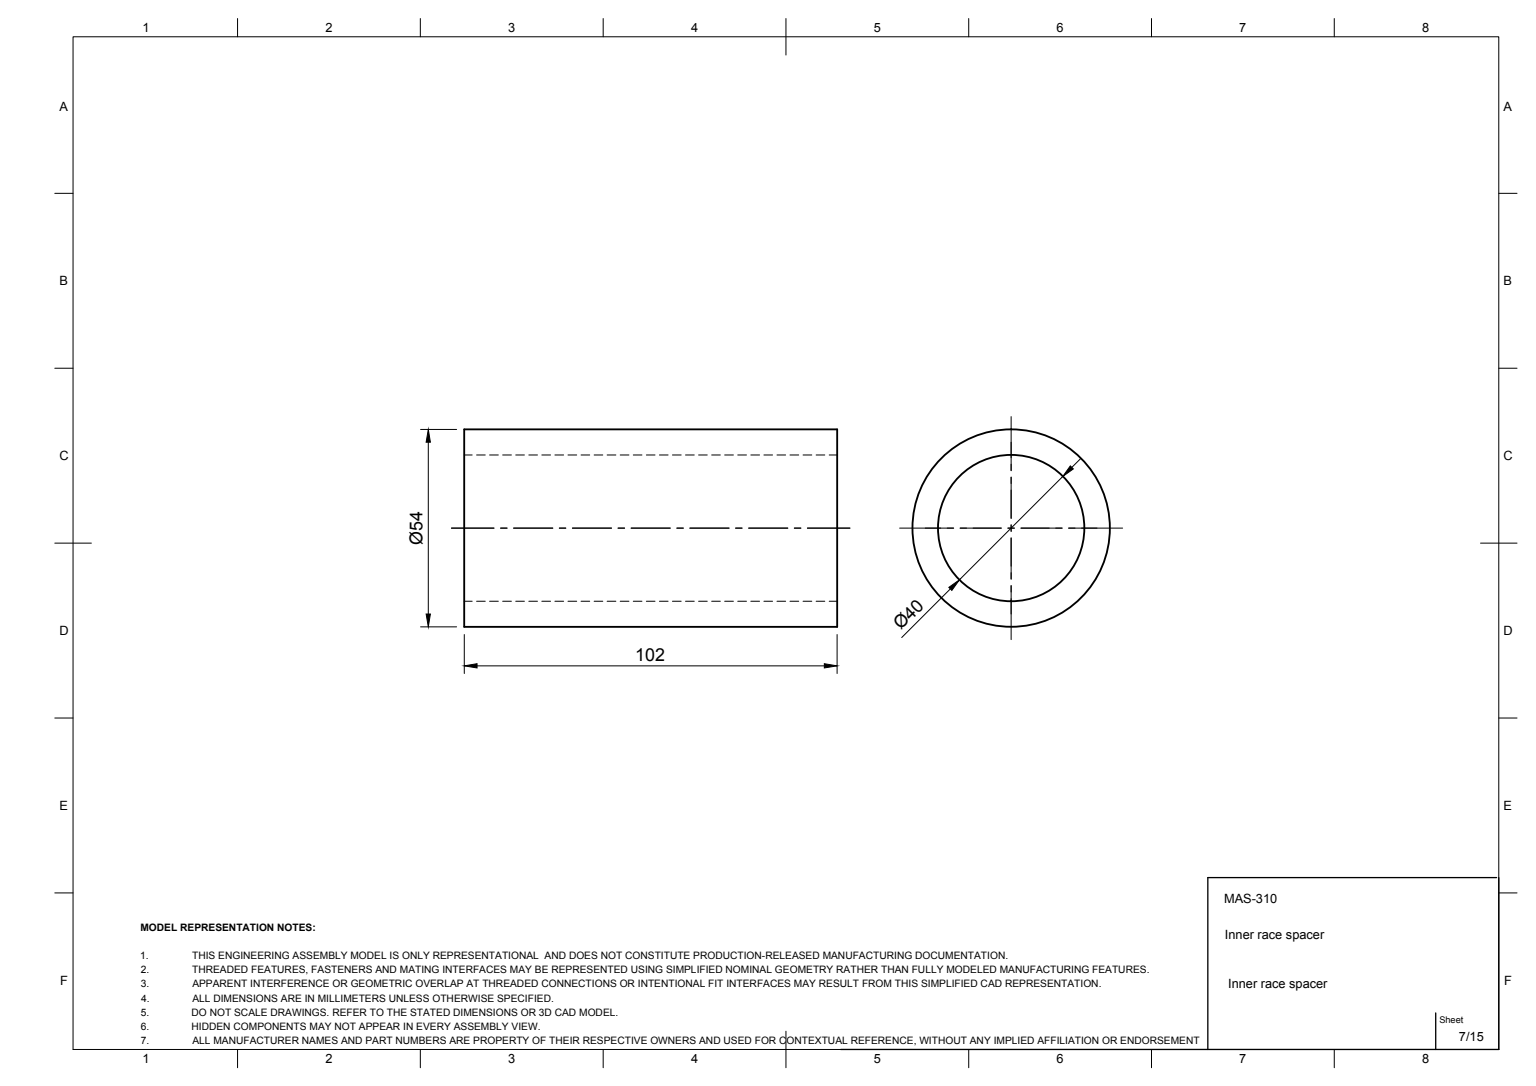
ISO-10303-21;
HEADER;
/* Generated by software containing ST-Developer
 * from STEP Tools, Inc. (www.steptools.com) 
 */

FILE_DESCRIPTION(
/* description */ ('Independent30mm screw-fed quill/spindle unit with16mm straight tool s
ocket, radial set screw, native reusable open ball bearings, retained 
inner/outer race stacks, keyed quill guide and M12x1.75 fine feed. Ext
ernal moving drive and tool not included. Ideal cage orbital links; in
dividual ball spin, force and preload not simulated. No drilling capac
ity, runout, speed, torque, load, life or machine safety rating.'),
/* implementation_level */ '2;1');

FILE_NAME(
/* name */ 'Inner race spacer.step',
/* time_stamp */ '2026-11-08T18:59:42-08:00',
/* author */ (''),
/* organization */ (''),
/* preprocessor_version */ 'ST-DEVELOPER v20.2',
/* originating_system */ 'Autodesk Translation Framework v15.17.0.0',
/* authorisation */ '');

FILE_SCHEMA (('AUTOMOTIVE_DESIGN { 1 0 10303 214 3 1 1 }'));
ENDSEC;

DATA;
#10=MECHANICAL_DESIGN_GEOMETRIC_PRESENTATION_REPRESENTATION('',(#1595),#63898);
#1559=SHAPE_REPRESENTATION_RELATIONSHIP('SRR','None',#63998,#1577);
#1577=ADVANCED_BREP_SHAPE_REPRESENTATION('',(#1613),#63883);
#1595=STYLED_ITEM('',(#64097),#1613);
#1613=MANIFOLD_SOLID_BREP('Body1',#15481);
#1669=FACE_BOUND('',#4012,.T.);
#1670=FACE_BOUND('',#4014,.T.);
#2106=CYLINDRICAL_SURFACE('',#16269,20.);
#2107=CYLINDRICAL_SURFACE('',#16272,27.);
#2499=CIRCLE('',#16270,20.);
#2500=CIRCLE('',#16271,20.);
#2501=CIRCLE('',#16273,27.);
#2502=CIRCLE('',#16274,27.);
#3130=FACE_OUTER_BOUND('',#4009,.T.);
#3131=FACE_OUTER_BOUND('',#4010,.T.);
#3132=FACE_OUTER_BOUND('',#4011,.T.);
#3133=FACE_OUTER_BOUND('',#4013,.T.);
#4009=EDGE_LOOP('',(#12496,#12497,#12498,#12499));
#4010=EDGE_LOOP('',(#12500,#12501,#12502,#12503));
#4011=EDGE_LOOP('',(#12504));
#4012=EDGE_LOOP('',(#12505));
#4013=EDGE_LOOP('',(#12506));
#4014=EDGE_LOOP('',(#12507));
#4856=LINE('',#46760,#5619);
#4857=LINE('',#46766,#5620);
#5619=VECTOR('',#18444,20.);
#5620=VECTOR('',#18451,27.);
#6832=VERTEX_POINT('',#46757);
#6833=VERTEX_POINT('',#46759);
#6834=VERTEX_POINT('',#46763);
#6835=VERTEX_POINT('',#46765);
#8837=EDGE_CURVE('',#6832,#6832,#2499,.T.);
#8838=EDGE_CURVE('',#6832,#6833,#4856,.T.);
#8839=EDGE_CURVE('',#6833,#6833,#2500,.T.);
#8840=EDGE_CURVE('',#6834,#6834,#2501,.T.);
#8841=EDGE_CURVE('',#6834,#6835,#4857,.T.);
#8842=EDGE_CURVE('',#6835,#6835,#2502,.T.);
#12496=ORIENTED_EDGE('',*,*,#8837,.F.);
#12497=ORIENTED_EDGE('',*,*,#8838,.T.);
#12498=ORIENTED_EDGE('',*,*,#8839,.T.);
#12499=ORIENTED_EDGE('',*,*,#8838,.F.);
#12500=ORIENTED_EDGE('',*,*,#8840,.F.);
#12501=ORIENTED_EDGE('',*,*,#8841,.T.);
#12502=ORIENTED_EDGE('',*,*,#8842,.T.);
#12503=ORIENTED_EDGE('',*,*,#8841,.F.);
#12504=ORIENTED_EDGE('',*,*,#8840,.T.);
#12505=ORIENTED_EDGE('',*,*,#8837,.T.);
#12506=ORIENTED_EDGE('',*,*,#8842,.F.);
#12507=ORIENTED_EDGE('',*,*,#8839,.F.);
#14569=PLANE('',#16275);
#14570=PLANE('',#16276);
#15110=ADVANCED_FACE('',(#3130),#2106,.F.);
#15111=ADVANCED_FACE('',(#3131),#2107,.T.);
#15112=ADVANCED_FACE('',(#3132,#1669),#14569,.T.);
#15113=ADVANCED_FACE('',(#3133,#1670),#14570,.F.);
#15481=CLOSED_SHELL('',(#15110,#15111,#15112,#15113));
#16268=AXIS2_PLACEMENT_3D('',#46755,#18438,#18439);
#16269=AXIS2_PLACEMENT_3D('',#46756,#18440,#18441);
#16270=AXIS2_PLACEMENT_3D('',#46758,#18442,#18443);
#16271=AXIS2_PLACEMENT_3D('',#46761,#18445,#18446);
#16272=AXIS2_PLACEMENT_3D('',#46762,#18447,#18448);
#16273=AXIS2_PLACEMENT_3D('',#46764,#18449,#18450);
#16274=AXIS2_PLACEMENT_3D('',#46767,#18452,#18453);
#16275=AXIS2_PLACEMENT_3D('',#46768,#18454,#18455);
#16276=AXIS2_PLACEMENT_3D('',#46769,#18456,#18457);
#18438=DIRECTION('axis',(0.,0.,1.));
#18439=DIRECTION('refdir',(1.,0.,0.));
#18440=DIRECTION('center_axis',(0.,0.,1.));
#18441=DIRECTION('ref_axis',(1.,0.,0.));
#18442=DIRECTION('center_axis',(0.,0.,-1.));
#18443=DIRECTION('ref_axis',(1.,0.,0.));
#18444=DIRECTION('',(0.,0.,-1.));
#18445=DIRECTION('center_axis',(0.,0.,-1.));
#18446=DIRECTION('ref_axis',(1.,0.,0.));
#18447=DIRECTION('center_axis',(0.,0.,1.));
#18448=DIRECTION('ref_axis',(1.,0.,0.));
#18449=DIRECTION('center_axis',(0.,0.,1.));
#18450=DIRECTION('ref_axis',(1.,0.,0.));
#18451=DIRECTION('',(0.,0.,-1.));
#18452=DIRECTION('center_axis',(0.,0.,1.));
#18453=DIRECTION('ref_axis',(1.,0.,0.));
#18454=DIRECTION('center_axis',(0.,0.,1.));
#18455=DIRECTION('ref_axis',(1.,0.,0.));
#18456=DIRECTION('center_axis',(0.,0.,1.));
#18457=DIRECTION('ref_axis',(1.,0.,0.));
#46755=CARTESIAN_POINT('',(0.,0.,0.));
#46756=CARTESIAN_POINT('Origin',(0.,0.,59.));
#46757=CARTESIAN_POINT('',(-20.,-2.44929359829471E-15,161.));
#46758=CARTESIAN_POINT('Origin',(0.,0.,161.));
#46759=CARTESIAN_POINT('',(-20.,-2.44929359829471E-15,59.));
#46760=CARTESIAN_POINT('',(-20.,-2.44929359829471E-15,59.));
#46761=CARTESIAN_POINT('Origin',(0.,0.,59.));
#46762=CARTESIAN_POINT('Origin',(0.,0.,59.));
#46763=CARTESIAN_POINT('',(-27.,-3.30654635769785E-15,161.));
#46764=CARTESIAN_POINT('Origin',(0.,0.,161.));
#46765=CARTESIAN_POINT('',(-27.,-3.30654635769785E-15,59.));
#46766=CARTESIAN_POINT('',(-27.,-3.30654635769785E-15,59.));
#46767=CARTESIAN_POINT('Origin',(0.,0.,59.));
#46768=CARTESIAN_POINT('Origin',(0.,0.,161.));
#46769=CARTESIAN_POINT('Origin',(0.,0.,59.));
#63863=UNCERTAINTY_MEASURE_WITH_UNIT(LENGTH_MEASURE(0.01),#63899,
'DISTANCE_ACCURACY_VALUE',
'Maximum model space distance between geometric entities at asserted c
onnectivities');
#63878=UNCERTAINTY_MEASURE_WITH_UNIT(LENGTH_MEASURE(0.01),#63899,
'DISTANCE_ACCURACY_VALUE',
'Maximum model space distance between geometric entities at asserted c
onnectivities');
#63883=(
GEOMETRIC_REPRESENTATION_CONTEXT(3)
GLOBAL_UNCERTAINTY_ASSIGNED_CONTEXT((#63863))
GLOBAL_UNIT_ASSIGNED_CONTEXT((#63899,#63901,#63902))
REPRESENTATION_CONTEXT('','3D')
);
#63898=(
GEOMETRIC_REPRESENTATION_CONTEXT(3)
GLOBAL_UNCERTAINTY_ASSIGNED_CONTEXT((#63878))
GLOBAL_UNIT_ASSIGNED_CONTEXT((#63899,#63901,#63902))
REPRESENTATION_CONTEXT('','3D')
);
#63899=(
LENGTH_UNIT()
NAMED_UNIT(*)
SI_UNIT(.MILLI.,.METRE.)
);
#63901=(
NAMED_UNIT(*)
PLANE_ANGLE_UNIT()
SI_UNIT($,.RADIAN.)
);
#63902=(
NAMED_UNIT(*)
SI_UNIT($,.STERADIAN.)
SOLID_ANGLE_UNIT()
);
#63907=SHAPE_DEFINITION_REPRESENTATION(#63926,#63998);
#63926=PRODUCT_DEFINITION_SHAPE('',$,#64018);
#63998=SHAPE_REPRESENTATION('',(#16268),#63883);
#64013=PRODUCT_DEFINITION_CONTEXT('part definition',#64072,'design');
#64018=PRODUCT_DEFINITION('Inner race spacer','Inner race spacer',#64037,
#64013);
#64037=PRODUCT_DEFINITION_FORMATION('',$,#64078);
#64072=APPLICATION_CONTEXT(
'Core Data for Automotive Mechanical Design Process');
#64073=PRODUCT_CONTEXT('part definition',#64072,'mechanical');
#64078=PRODUCT('Inner race spacer','Inner race spacer',
'Inner race spacer',(#64073));
#64097=PRESENTATION_STYLE_ASSIGNMENT((#64110));
#64110=SURFACE_STYLE_USAGE(.BOTH.,#64123);
#64123=SURFACE_SIDE_STYLE('',(#64136));
#64136=SURFACE_STYLE_FILL_AREA(#64149);
#64149=FILL_AREA_STYLE('Light gray',(#64162));
#64162=FILL_AREA_STYLE_COLOUR('Light gray',#64175);
#64175=COLOUR_RGB('Light gray',0.725490196078431,0.752941176470588,0.792156862745098);
ENDSEC;
END-ISO-10303-21;
